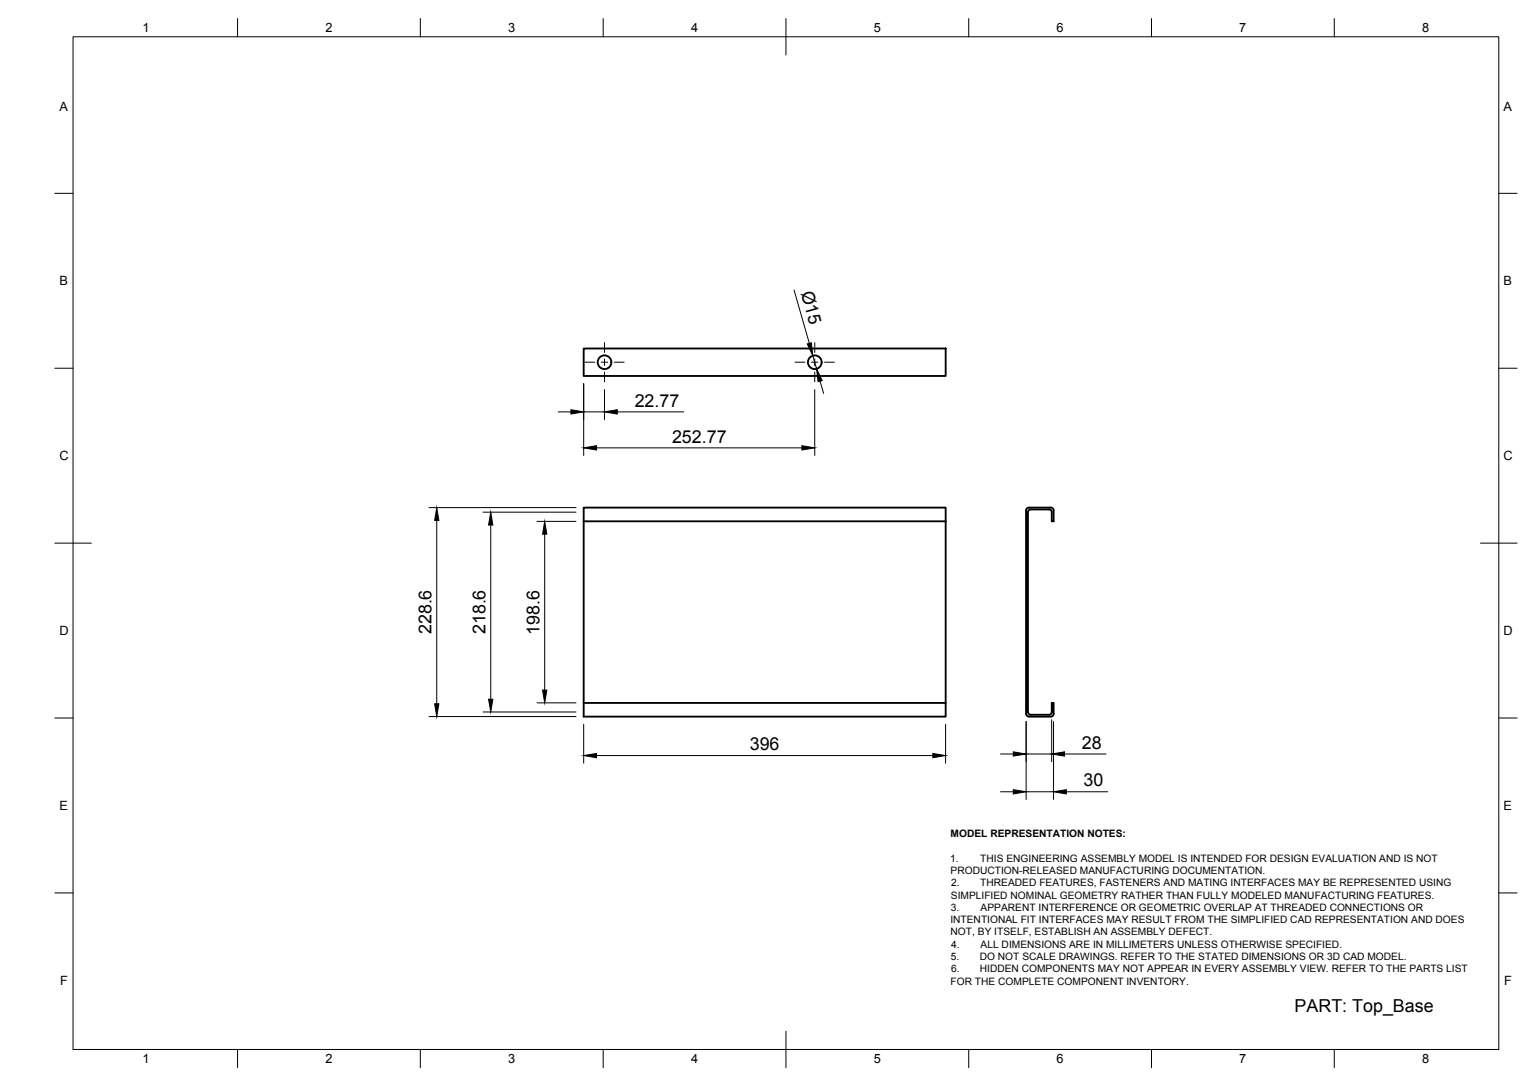
ISO-10303-21;
HEADER;
/* Generated by software containing ST-Developer
 * from STEP Tools, Inc. (www.steptools.com) 
 */

FILE_DESCRIPTION(
/* description */ (''),
/* implementation_level */ '2;1');

FILE_NAME(
/* name */ 'Top_Base.step',
/* time_stamp */ '2026-10-05T15:35:09-07:00',
/* author */ (''),
/* organization */ (''),
/* preprocessor_version */ 'ST-DEVELOPER v20.2',
/* originating_system */ 'Autodesk Translation Framework v15.15.0.0',
/* authorisation */ '');

FILE_SCHEMA (('AUTOMOTIVE_DESIGN { 1 0 10303 214 3 1 1 }'));
ENDSEC;

DATA;
#10=MECHANICAL_DESIGN_GEOMETRIC_PRESENTATION_REPRESENTATION('',(#548),#74523);
#530=SHAPE_REPRESENTATION_RELATIONSHIP('SRR','None',#74563,#539);
#539=ADVANCED_BREP_SHAPE_REPRESENTATION('',(#557),#74519);
#548=STYLED_ITEM('',(#74612),#557);
#557=MANIFOLD_SOLID_BREP('Body1',#4727);
#594=FACE_BOUND('',#944,.T.);
#595=FACE_BOUND('',#945,.T.);
#596=FACE_BOUND('',#949,.T.);
#597=FACE_BOUND('',#950,.T.);
#598=FACE_BOUND('',#958,.T.);
#599=FACE_BOUND('',#959,.T.);
#600=FACE_BOUND('',#965,.T.);
#601=FACE_BOUND('',#966,.T.);
#649=PLANE('',#4999);
#650=PLANE('',#5000);
#651=PLANE('',#5004);
#652=PLANE('',#5011);
#653=PLANE('',#5015);
#654=PLANE('',#5016);
#655=PLANE('',#5021);
#656=PLANE('',#5022);
#657=PLANE('',#5025);
#658=PLANE('',#5028);
#659=PLANE('',#5029);
#660=PLANE('',#5032);
#661=PLANE('',#5035);
#662=PLANE('',#5036);
#759=FACE_OUTER_BOUND('',#936,.T.);
#760=FACE_OUTER_BOUND('',#937,.T.);
#761=FACE_OUTER_BOUND('',#938,.T.);
#762=FACE_OUTER_BOUND('',#939,.T.);
#763=FACE_OUTER_BOUND('',#940,.T.);
#764=FACE_OUTER_BOUND('',#941,.T.);
#765=FACE_OUTER_BOUND('',#942,.T.);
#766=FACE_OUTER_BOUND('',#943,.T.);
#767=FACE_OUTER_BOUND('',#946,.T.);
#768=FACE_OUTER_BOUND('',#947,.T.);
#769=FACE_OUTER_BOUND('',#948,.T.);
#770=FACE_OUTER_BOUND('',#951,.T.);
#771=FACE_OUTER_BOUND('',#952,.T.);
#772=FACE_OUTER_BOUND('',#953,.T.);
#773=FACE_OUTER_BOUND('',#954,.T.);
#774=FACE_OUTER_BOUND('',#955,.T.);
#775=FACE_OUTER_BOUND('',#956,.T.);
#776=FACE_OUTER_BOUND('',#957,.T.);
#777=FACE_OUTER_BOUND('',#960,.T.);
#778=FACE_OUTER_BOUND('',#961,.T.);
#779=FACE_OUTER_BOUND('',#962,.T.);
#780=FACE_OUTER_BOUND('',#963,.T.);
#781=FACE_OUTER_BOUND('',#964,.T.);
#782=FACE_OUTER_BOUND('',#967,.T.);
#783=FACE_OUTER_BOUND('',#968,.T.);
#784=FACE_OUTER_BOUND('',#969,.T.);
#936=EDGE_LOOP('',(#3332,#3333,#3334,#3335));
#937=EDGE_LOOP('',(#3336,#3337,#3338,#3339));
#938=EDGE_LOOP('',(#3340,#3341,#3342,#3343));
#939=EDGE_LOOP('',(#3344,#3345,#3346,#3347));
#940=EDGE_LOOP('',(#3348,#3349,#3350,#3351));
#941=EDGE_LOOP('',(#3352,#3353,#3354,#3355));
#942=EDGE_LOOP('',(#3356,#3357,#3358,#3359));
#943=EDGE_LOOP('',(#3360,#3361,#3362,#3363));
#944=EDGE_LOOP('',(#3364));
#945=EDGE_LOOP('',(#3365));
#946=EDGE_LOOP('',(#3366,#3367,#3368,#3369));
#947=EDGE_LOOP('',(#3370,#3371,#3372,#3373));
#948=EDGE_LOOP('',(#3374,#3375,#3376,#3377));
#949=EDGE_LOOP('',(#3378));
#950=EDGE_LOOP('',(#3379));
#951=EDGE_LOOP('',(#3380,#3381,#3382,#3383));
#952=EDGE_LOOP('',(#3384,#3385,#3386,#3387));
#953=EDGE_LOOP('',(#3388,#3389,#3390,#3391,#3392,#3393,#3394,#3395,#3396,
#3397,#3398,#3399,#3400,#3401,#3402,#3403,#3404,#3405,#3406,#3407));
#954=EDGE_LOOP('',(#3408,#3409,#3410,#3411));
#955=EDGE_LOOP('',(#3412,#3413,#3414,#3415));
#956=EDGE_LOOP('',(#3416,#3417,#3418,#3419));
#957=EDGE_LOOP('',(#3420,#3421,#3422,#3423));
#958=EDGE_LOOP('',(#3424));
#959=EDGE_LOOP('',(#3425));
#960=EDGE_LOOP('',(#3426,#3427,#3428,#3429));
#961=EDGE_LOOP('',(#3430,#3431,#3432,#3433));
#962=EDGE_LOOP('',(#3434,#3435,#3436,#3437));
#963=EDGE_LOOP('',(#3438,#3439,#3440,#3441));
#964=EDGE_LOOP('',(#3442,#3443,#3444,#3445));
#965=EDGE_LOOP('',(#3446));
#966=EDGE_LOOP('',(#3447));
#967=EDGE_LOOP('',(#3448,#3449,#3450,#3451));
#968=EDGE_LOOP('',(#3452,#3453,#3454,#3455));
#969=EDGE_LOOP('',(#3456,#3457,#3458,#3459,#3460,#3461,#3462,#3463,#3464,
#3465,#3466,#3467,#3468,#3469,#3470,#3471,#3472,#3473,#3474,#3475));
#1128=LINE('',#6314,#1325);
#1129=LINE('',#6320,#1326);
#1130=LINE('',#6326,#1327);
#1131=LINE('',#6332,#1328);
#1132=LINE('',#6337,#1329);
#1133=LINE('',#6339,#1330);
#1134=LINE('',#6341,#1331);
#1135=LINE('',#6342,#1332);
#1136=LINE('',#6345,#1333);
#1137=LINE('',#6347,#1334);
#1138=LINE('',#6348,#1335);
#1139=LINE('',#6353,#1336);
#1140=LINE('',#6357,#1337);
#1141=LINE('',#6359,#1338);
#1142=LINE('',#6360,#1339);
#1143=LINE('',#6365,#1340);
#1144=LINE('',#6370,#1341);
#1145=LINE('',#6374,#1342);
#1146=LINE('',#6378,#1343);
#1147=LINE('',#6380,#1344);
#1148=LINE('',#6381,#1345);
#1149=LINE('',#6386,#1346);
#1150=LINE('',#6389,#1347);
#1151=LINE('',#6390,#1348);
#1152=LINE('',#6394,#1349);
#1153=LINE('',#6396,#1350);
#1154=LINE('',#6398,#1351);
#1155=LINE('',#6402,#1352);
#1156=LINE('',#6405,#1353);
#1157=LINE('',#6407,#1354);
#1158=LINE('',#6411,#1355);
#1159=LINE('',#6415,#1356);
#1160=LINE('',#6417,#1357);
#1161=LINE('',#6418,#1358);
#1162=LINE('',#6421,#1359);
#1163=LINE('',#6422,#1360);
#1164=LINE('',#6426,#1361);
#1165=LINE('',#6429,#1362);
#1166=LINE('',#6430,#1363);
#1167=LINE('',#6434,#1364);
#1168=LINE('',#6436,#1365);
#1169=LINE('',#6439,#1366);
#1170=LINE('',#6440,#1367);
#1171=LINE('',#6444,#1368);
#1172=LINE('',#6447,#1369);
#1173=LINE('',#6448,#1370);
#1174=LINE('',#6452,#1371);
#1175=LINE('',#6454,#1372);
#1325=VECTOR('',#5524,7.5);
#1326=VECTOR('',#5531,7.5);
#1327=VECTOR('',#5538,7.5);
#1328=VECTOR('',#5545,7.5);
#1329=VECTOR('',#5550,10.);
#1330=VECTOR('',#5551,10.);
#1331=VECTOR('',#5552,10.);
#1332=VECTOR('',#5553,10.);
#1333=VECTOR('',#5556,10.);
#1334=VECTOR('',#5557,10.);
#1335=VECTOR('',#5558,10.);
#1336=VECTOR('',#5563,10.);
#1337=VECTOR('',#5568,10.);
#1338=VECTOR('',#5569,10.);
#1339=VECTOR('',#5570,10.);
#1340=VECTOR('',#5575,10.);
#1341=VECTOR('',#5580,10.);
#1342=VECTOR('',#5583,10.);
#1343=VECTOR('',#5588,10.);
#1344=VECTOR('',#5589,10.);
#1345=VECTOR('',#5590,10.);
#1346=VECTOR('',#5595,10.);
#1347=VECTOR('',#5600,10.);
#1348=VECTOR('',#5601,10.);
#1349=VECTOR('',#5604,10.);
#1350=VECTOR('',#5605,10.);
#1351=VECTOR('',#5606,10.);
#1352=VECTOR('',#5609,10.);
#1353=VECTOR('',#5612,10.);
#1354=VECTOR('',#5613,10.);
#1355=VECTOR('',#5616,10.);
#1356=VECTOR('',#5621,10.);
#1357=VECTOR('',#5622,10.);
#1358=VECTOR('',#5623,10.);
#1359=VECTOR('',#5626,10.);
#1360=VECTOR('',#5627,10.);
#1361=VECTOR('',#5632,10.);
#1362=VECTOR('',#5635,10.);
#1363=VECTOR('',#5636,10.);
#1364=VECTOR('',#5641,10.);
#1365=VECTOR('',#5644,10.);
#1366=VECTOR('',#5647,10.);
#1367=VECTOR('',#5648,10.);
#1368=VECTOR('',#5653,10.);
#1369=VECTOR('',#5656,10.);
#1370=VECTOR('',#5657,10.);
#1371=VECTOR('',#5662,10.);
#1372=VECTOR('',#5665,10.);
#1484=CIRCLE('',#4988,7.5);
#1485=CIRCLE('',#4989,7.5);
#1486=CIRCLE('',#4991,7.5);
#1487=CIRCLE('',#4992,7.5);
#1488=CIRCLE('',#4994,7.5);
#1489=CIRCLE('',#4995,7.5);
#1490=CIRCLE('',#4997,7.5);
#1491=CIRCLE('',#4998,7.5);
#1492=CIRCLE('',#5002,3.00000000000002);
#1493=CIRCLE('',#5003,3.00000000000002);
#1494=CIRCLE('',#5006,3.00000000000002);
#1495=CIRCLE('',#5007,3.00000000000002);
#1496=CIRCLE('',#5009,3.00000000000002);
#1497=CIRCLE('',#5010,3.00000000000002);
#1498=CIRCLE('',#5013,3.00000000000002);
#1499=CIRCLE('',#5014,3.00000000000002);
#1500=CIRCLE('',#5017,3.00000000000002);
#1501=CIRCLE('',#5018,3.00000000000002);
#1502=CIRCLE('',#5019,3.00000000000002);
#1503=CIRCLE('',#5020,3.00000000000002);
#1504=CIRCLE('',#5024,3.00000000000002);
#1505=CIRCLE('',#5027,3.00000000000002);
#1506=CIRCLE('',#5031,3.00000000000002);
#1507=CIRCLE('',#5034,3.00000000000002);
#1647=VERTEX_POINT('',#6311);
#1648=VERTEX_POINT('',#6313);
#1649=VERTEX_POINT('',#6317);
#1650=VERTEX_POINT('',#6319);
#1651=VERTEX_POINT('',#6323);
#1652=VERTEX_POINT('',#6325);
#1653=VERTEX_POINT('',#6329);
#1654=VERTEX_POINT('',#6331);
#1655=VERTEX_POINT('',#6335);
#1656=VERTEX_POINT('',#6336);
#1657=VERTEX_POINT('',#6338);
#1658=VERTEX_POINT('',#6340);
#1659=VERTEX_POINT('',#6344);
#1660=VERTEX_POINT('',#6346);
#1661=VERTEX_POINT('',#6350);
#1662=VERTEX_POINT('',#6352);
#1663=VERTEX_POINT('',#6356);
#1664=VERTEX_POINT('',#6358);
#1665=VERTEX_POINT('',#6362);
#1666=VERTEX_POINT('',#6364);
#1667=VERTEX_POINT('',#6368);
#1668=VERTEX_POINT('',#6369);
#1669=VERTEX_POINT('',#6371);
#1670=VERTEX_POINT('',#6373);
#1671=VERTEX_POINT('',#6377);
#1672=VERTEX_POINT('',#6379);
#1673=VERTEX_POINT('',#6383);
#1674=VERTEX_POINT('',#6385);
#1675=VERTEX_POINT('',#6392);
#1676=VERTEX_POINT('',#6393);
#1677=VERTEX_POINT('',#6395);
#1678=VERTEX_POINT('',#6397);
#1679=VERTEX_POINT('',#6399);
#1680=VERTEX_POINT('',#6401);
#1681=VERTEX_POINT('',#6403);
#1682=VERTEX_POINT('',#6406);
#1683=VERTEX_POINT('',#6408);
#1684=VERTEX_POINT('',#6410);
#1685=VERTEX_POINT('',#6414);
#1686=VERTEX_POINT('',#6416);
#1687=VERTEX_POINT('',#6420);
#1688=VERTEX_POINT('',#6424);
#1689=VERTEX_POINT('',#6428);
#1690=VERTEX_POINT('',#6432);
#1691=VERTEX_POINT('',#6438);
#1692=VERTEX_POINT('',#6442);
#1693=VERTEX_POINT('',#6446);
#1694=VERTEX_POINT('',#6450);
#2367=EDGE_CURVE('',#1647,#1647,#1484,.T.);
#2368=EDGE_CURVE('',#1647,#1648,#1128,.T.);
#2369=EDGE_CURVE('',#1648,#1648,#1485,.T.);
#2370=EDGE_CURVE('',#1649,#1649,#1486,.T.);
#2371=EDGE_CURVE('',#1649,#1650,#1129,.T.);
#2372=EDGE_CURVE('',#1650,#1650,#1487,.T.);
#2373=EDGE_CURVE('',#1651,#1651,#1488,.T.);
#2374=EDGE_CURVE('',#1651,#1652,#1130,.T.);
#2375=EDGE_CURVE('',#1652,#1652,#1489,.T.);
#2376=EDGE_CURVE('',#1653,#1653,#1490,.T.);
#2377=EDGE_CURVE('',#1653,#1654,#1131,.T.);
#2378=EDGE_CURVE('',#1654,#1654,#1491,.T.);
#2379=EDGE_CURVE('',#1655,#1656,#1132,.T.);
#2380=EDGE_CURVE('',#1656,#1657,#1133,.T.);
#2381=EDGE_CURVE('',#1657,#1658,#1134,.T.);
#2382=EDGE_CURVE('',#1658,#1655,#1135,.T.);
#2383=EDGE_CURVE('',#1657,#1659,#1136,.T.);
#2384=EDGE_CURVE('',#1659,#1660,#1137,.T.);
#2385=EDGE_CURVE('',#1660,#1658,#1138,.T.);
#2386=EDGE_CURVE('',#1659,#1661,#1492,.T.);
#2387=EDGE_CURVE('',#1661,#1662,#1139,.T.);
#2388=EDGE_CURVE('',#1662,#1660,#1493,.T.);
#2389=EDGE_CURVE('',#1661,#1663,#1140,.T.);
#2390=EDGE_CURVE('',#1663,#1664,#1141,.T.);
#2391=EDGE_CURVE('',#1664,#1662,#1142,.T.);
#2392=EDGE_CURVE('',#1663,#1665,#1494,.T.);
#2393=EDGE_CURVE('',#1665,#1666,#1143,.T.);
#2394=EDGE_CURVE('',#1666,#1664,#1495,.T.);
#2395=EDGE_CURVE('',#1667,#1668,#1144,.T.);
#2396=EDGE_CURVE('',#1667,#1669,#1496,.T.);
#2397=EDGE_CURVE('',#1669,#1670,#1145,.T.);
#2398=EDGE_CURVE('',#1670,#1668,#1497,.T.);
#2399=EDGE_CURVE('',#1669,#1671,#1146,.T.);
#2400=EDGE_CURVE('',#1671,#1672,#1147,.T.);
#2401=EDGE_CURVE('',#1672,#1670,#1148,.T.);
#2402=EDGE_CURVE('',#1671,#1673,#1498,.T.);
#2403=EDGE_CURVE('',#1673,#1674,#1149,.T.);
#2404=EDGE_CURVE('',#1674,#1672,#1499,.T.);
#2405=EDGE_CURVE('',#1673,#1656,#1150,.T.);
#2406=EDGE_CURVE('',#1655,#1674,#1151,.T.);
#2407=EDGE_CURVE('',#1675,#1676,#1152,.T.);
#2408=EDGE_CURVE('',#1676,#1677,#1153,.T.);
#2409=EDGE_CURVE('',#1677,#1678,#1154,.T.);
#2410=EDGE_CURVE('',#1678,#1679,#1500,.T.);
#2411=EDGE_CURVE('',#1679,#1680,#1155,.T.);
#2412=EDGE_CURVE('',#1680,#1681,#1501,.T.);
#2413=EDGE_CURVE('',#1681,#1665,#1156,.T.);
#2414=EDGE_CURVE('',#1682,#1667,#1157,.T.);
#2415=EDGE_CURVE('',#1682,#1683,#1502,.T.);
#2416=EDGE_CURVE('',#1683,#1684,#1158,.T.);
#2417=EDGE_CURVE('',#1684,#1675,#1503,.T.);
#2418=EDGE_CURVE('',#1685,#1676,#1159,.T.);
#2419=EDGE_CURVE('',#1686,#1685,#1160,.T.);
#2420=EDGE_CURVE('',#1677,#1686,#1161,.T.);
#2421=EDGE_CURVE('',#1687,#1686,#1162,.T.);
#2422=EDGE_CURVE('',#1678,#1687,#1163,.T.);
#2423=EDGE_CURVE('',#1688,#1687,#1504,.T.);
#2424=EDGE_CURVE('',#1679,#1688,#1164,.T.);
#2425=EDGE_CURVE('',#1689,#1688,#1165,.T.);
#2426=EDGE_CURVE('',#1680,#1689,#1166,.T.);
#2427=EDGE_CURVE('',#1690,#1689,#1505,.T.);
#2428=EDGE_CURVE('',#1681,#1690,#1167,.T.);
#2429=EDGE_CURVE('',#1690,#1666,#1168,.T.);
#2430=EDGE_CURVE('',#1691,#1668,#1169,.T.);
#2431=EDGE_CURVE('',#1682,#1691,#1170,.T.);
#2432=EDGE_CURVE('',#1692,#1691,#1506,.T.);
#2433=EDGE_CURVE('',#1683,#1692,#1171,.T.);
#2434=EDGE_CURVE('',#1693,#1692,#1172,.T.);
#2435=EDGE_CURVE('',#1684,#1693,#1173,.T.);
#2436=EDGE_CURVE('',#1694,#1693,#1507,.T.);
#2437=EDGE_CURVE('',#1675,#1694,#1174,.T.);
#2438=EDGE_CURVE('',#1685,#1694,#1175,.T.);
#3332=ORIENTED_EDGE('',*,*,#2367,.F.);
#3333=ORIENTED_EDGE('',*,*,#2368,.T.);
#3334=ORIENTED_EDGE('',*,*,#2369,.F.);
#3335=ORIENTED_EDGE('',*,*,#2368,.F.);
#3336=ORIENTED_EDGE('',*,*,#2370,.F.);
#3337=ORIENTED_EDGE('',*,*,#2371,.T.);
#3338=ORIENTED_EDGE('',*,*,#2372,.F.);
#3339=ORIENTED_EDGE('',*,*,#2371,.F.);
#3340=ORIENTED_EDGE('',*,*,#2373,.F.);
#3341=ORIENTED_EDGE('',*,*,#2374,.T.);
#3342=ORIENTED_EDGE('',*,*,#2375,.F.);
#3343=ORIENTED_EDGE('',*,*,#2374,.F.);
#3344=ORIENTED_EDGE('',*,*,#2376,.F.);
#3345=ORIENTED_EDGE('',*,*,#2377,.T.);
#3346=ORIENTED_EDGE('',*,*,#2378,.F.);
#3347=ORIENTED_EDGE('',*,*,#2377,.F.);
#3348=ORIENTED_EDGE('',*,*,#2379,.T.);
#3349=ORIENTED_EDGE('',*,*,#2380,.T.);
#3350=ORIENTED_EDGE('',*,*,#2381,.T.);
#3351=ORIENTED_EDGE('',*,*,#2382,.T.);
#3352=ORIENTED_EDGE('',*,*,#2381,.F.);
#3353=ORIENTED_EDGE('',*,*,#2383,.T.);
#3354=ORIENTED_EDGE('',*,*,#2384,.T.);
#3355=ORIENTED_EDGE('',*,*,#2385,.T.);
#3356=ORIENTED_EDGE('',*,*,#2384,.F.);
#3357=ORIENTED_EDGE('',*,*,#2386,.T.);
#3358=ORIENTED_EDGE('',*,*,#2387,.T.);
#3359=ORIENTED_EDGE('',*,*,#2388,.T.);
#3360=ORIENTED_EDGE('',*,*,#2387,.F.);
#3361=ORIENTED_EDGE('',*,*,#2389,.T.);
#3362=ORIENTED_EDGE('',*,*,#2390,.T.);
#3363=ORIENTED_EDGE('',*,*,#2391,.T.);
#3364=ORIENTED_EDGE('',*,*,#2370,.T.);
#3365=ORIENTED_EDGE('',*,*,#2376,.T.);
#3366=ORIENTED_EDGE('',*,*,#2390,.F.);
#3367=ORIENTED_EDGE('',*,*,#2392,.T.);
#3368=ORIENTED_EDGE('',*,*,#2393,.T.);
#3369=ORIENTED_EDGE('',*,*,#2394,.T.);
#3370=ORIENTED_EDGE('',*,*,#2395,.F.);
#3371=ORIENTED_EDGE('',*,*,#2396,.T.);
#3372=ORIENTED_EDGE('',*,*,#2397,.T.);
#3373=ORIENTED_EDGE('',*,*,#2398,.T.);
#3374=ORIENTED_EDGE('',*,*,#2397,.F.);
#3375=ORIENTED_EDGE('',*,*,#2399,.T.);
#3376=ORIENTED_EDGE('',*,*,#2400,.T.);
#3377=ORIENTED_EDGE('',*,*,#2401,.T.);
#3378=ORIENTED_EDGE('',*,*,#2372,.T.);
#3379=ORIENTED_EDGE('',*,*,#2378,.T.);
#3380=ORIENTED_EDGE('',*,*,#2400,.F.);
#3381=ORIENTED_EDGE('',*,*,#2402,.T.);
#3382=ORIENTED_EDGE('',*,*,#2403,.T.);
#3383=ORIENTED_EDGE('',*,*,#2404,.T.);
#3384=ORIENTED_EDGE('',*,*,#2403,.F.);
#3385=ORIENTED_EDGE('',*,*,#2405,.T.);
#3386=ORIENTED_EDGE('',*,*,#2379,.F.);
#3387=ORIENTED_EDGE('',*,*,#2406,.T.);
#3388=ORIENTED_EDGE('',*,*,#2407,.T.);
#3389=ORIENTED_EDGE('',*,*,#2408,.T.);
#3390=ORIENTED_EDGE('',*,*,#2409,.T.);
#3391=ORIENTED_EDGE('',*,*,#2410,.T.);
#3392=ORIENTED_EDGE('',*,*,#2411,.T.);
#3393=ORIENTED_EDGE('',*,*,#2412,.T.);
#3394=ORIENTED_EDGE('',*,*,#2413,.T.);
#3395=ORIENTED_EDGE('',*,*,#2392,.F.);
#3396=ORIENTED_EDGE('',*,*,#2389,.F.);
#3397=ORIENTED_EDGE('',*,*,#2386,.F.);
#3398=ORIENTED_EDGE('',*,*,#2383,.F.);
#3399=ORIENTED_EDGE('',*,*,#2380,.F.);
#3400=ORIENTED_EDGE('',*,*,#2405,.F.);
#3401=ORIENTED_EDGE('',*,*,#2402,.F.);
#3402=ORIENTED_EDGE('',*,*,#2399,.F.);
#3403=ORIENTED_EDGE('',*,*,#2396,.F.);
#3404=ORIENTED_EDGE('',*,*,#2414,.F.);
#3405=ORIENTED_EDGE('',*,*,#2415,.T.);
#3406=ORIENTED_EDGE('',*,*,#2416,.T.);
#3407=ORIENTED_EDGE('',*,*,#2417,.T.);
#3408=ORIENTED_EDGE('',*,*,#2418,.F.);
#3409=ORIENTED_EDGE('',*,*,#2419,.F.);
#3410=ORIENTED_EDGE('',*,*,#2420,.F.);
#3411=ORIENTED_EDGE('',*,*,#2408,.F.);
#3412=ORIENTED_EDGE('',*,*,#2420,.T.);
#3413=ORIENTED_EDGE('',*,*,#2421,.F.);
#3414=ORIENTED_EDGE('',*,*,#2422,.F.);
#3415=ORIENTED_EDGE('',*,*,#2409,.F.);
#3416=ORIENTED_EDGE('',*,*,#2422,.T.);
#3417=ORIENTED_EDGE('',*,*,#2423,.F.);
#3418=ORIENTED_EDGE('',*,*,#2424,.F.);
#3419=ORIENTED_EDGE('',*,*,#2410,.F.);
#3420=ORIENTED_EDGE('',*,*,#2424,.T.);
#3421=ORIENTED_EDGE('',*,*,#2425,.F.);
#3422=ORIENTED_EDGE('',*,*,#2426,.F.);
#3423=ORIENTED_EDGE('',*,*,#2411,.F.);
#3424=ORIENTED_EDGE('',*,*,#2369,.T.);
#3425=ORIENTED_EDGE('',*,*,#2375,.T.);
#3426=ORIENTED_EDGE('',*,*,#2426,.T.);
#3427=ORIENTED_EDGE('',*,*,#2427,.F.);
#3428=ORIENTED_EDGE('',*,*,#2428,.F.);
#3429=ORIENTED_EDGE('',*,*,#2412,.F.);
#3430=ORIENTED_EDGE('',*,*,#2428,.T.);
#3431=ORIENTED_EDGE('',*,*,#2429,.T.);
#3432=ORIENTED_EDGE('',*,*,#2393,.F.);
#3433=ORIENTED_EDGE('',*,*,#2413,.F.);
#3434=ORIENTED_EDGE('',*,*,#2430,.F.);
#3435=ORIENTED_EDGE('',*,*,#2431,.F.);
#3436=ORIENTED_EDGE('',*,*,#2414,.T.);
#3437=ORIENTED_EDGE('',*,*,#2395,.T.);
#3438=ORIENTED_EDGE('',*,*,#2431,.T.);
#3439=ORIENTED_EDGE('',*,*,#2432,.F.);
#3440=ORIENTED_EDGE('',*,*,#2433,.F.);
#3441=ORIENTED_EDGE('',*,*,#2415,.F.);
#3442=ORIENTED_EDGE('',*,*,#2433,.T.);
#3443=ORIENTED_EDGE('',*,*,#2434,.F.);
#3444=ORIENTED_EDGE('',*,*,#2435,.F.);
#3445=ORIENTED_EDGE('',*,*,#2416,.F.);
#3446=ORIENTED_EDGE('',*,*,#2367,.T.);
#3447=ORIENTED_EDGE('',*,*,#2373,.T.);
#3448=ORIENTED_EDGE('',*,*,#2435,.T.);
#3449=ORIENTED_EDGE('',*,*,#2436,.F.);
#3450=ORIENTED_EDGE('',*,*,#2437,.F.);
#3451=ORIENTED_EDGE('',*,*,#2417,.F.);
#3452=ORIENTED_EDGE('',*,*,#2437,.T.);
#3453=ORIENTED_EDGE('',*,*,#2438,.F.);
#3454=ORIENTED_EDGE('',*,*,#2418,.T.);
#3455=ORIENTED_EDGE('',*,*,#2407,.F.);
#3456=ORIENTED_EDGE('',*,*,#2438,.T.);
#3457=ORIENTED_EDGE('',*,*,#2436,.T.);
#3458=ORIENTED_EDGE('',*,*,#2434,.T.);
#3459=ORIENTED_EDGE('',*,*,#2432,.T.);
#3460=ORIENTED_EDGE('',*,*,#2430,.T.);
#3461=ORIENTED_EDGE('',*,*,#2398,.F.);
#3462=ORIENTED_EDGE('',*,*,#2401,.F.);
#3463=ORIENTED_EDGE('',*,*,#2404,.F.);
#3464=ORIENTED_EDGE('',*,*,#2406,.F.);
#3465=ORIENTED_EDGE('',*,*,#2382,.F.);
#3466=ORIENTED_EDGE('',*,*,#2385,.F.);
#3467=ORIENTED_EDGE('',*,*,#2388,.F.);
#3468=ORIENTED_EDGE('',*,*,#2391,.F.);
#3469=ORIENTED_EDGE('',*,*,#2394,.F.);
#3470=ORIENTED_EDGE('',*,*,#2429,.F.);
#3471=ORIENTED_EDGE('',*,*,#2427,.T.);
#3472=ORIENTED_EDGE('',*,*,#2425,.T.);
#3473=ORIENTED_EDGE('',*,*,#2423,.T.);
#3474=ORIENTED_EDGE('',*,*,#2421,.T.);
#3475=ORIENTED_EDGE('',*,*,#2419,.T.);
#4551=CYLINDRICAL_SURFACE('',#4987,7.5);
#4552=CYLINDRICAL_SURFACE('',#4990,7.5);
#4553=CYLINDRICAL_SURFACE('',#4993,7.5);
#4554=CYLINDRICAL_SURFACE('',#4996,7.5);
#4555=CYLINDRICAL_SURFACE('',#5001,3.00000000000002);
#4556=CYLINDRICAL_SURFACE('',#5005,3.00000000000002);
#4557=CYLINDRICAL_SURFACE('',#5008,3.00000000000002);
#4558=CYLINDRICAL_SURFACE('',#5012,3.00000000000002);
#4559=CYLINDRICAL_SURFACE('',#5023,3.00000000000002);
#4560=CYLINDRICAL_SURFACE('',#5026,3.00000000000002);
#4561=CYLINDRICAL_SURFACE('',#5030,3.00000000000002);
#4562=CYLINDRICAL_SURFACE('',#5033,3.00000000000002);
#4655=ADVANCED_FACE('',(#759),#4551,.F.);
#4656=ADVANCED_FACE('',(#760),#4552,.F.);
#4657=ADVANCED_FACE('',(#761),#4553,.F.);
#4658=ADVANCED_FACE('',(#762),#4554,.F.);
#4659=ADVANCED_FACE('',(#763),#649,.F.);
#4660=ADVANCED_FACE('',(#764),#650,.F.);
#4661=ADVANCED_FACE('',(#765),#4555,.F.);
#4662=ADVANCED_FACE('',(#766,#594,#595),#651,.F.);
#4663=ADVANCED_FACE('',(#767),#4556,.F.);
#4664=ADVANCED_FACE('',(#768),#4557,.T.);
#4665=ADVANCED_FACE('',(#769,#596,#597),#652,.F.);
#4666=ADVANCED_FACE('',(#770),#4558,.T.);
#4667=ADVANCED_FACE('',(#771),#653,.F.);
#4668=ADVANCED_FACE('',(#772),#654,.F.);
#4669=ADVANCED_FACE('',(#773),#655,.T.);
#4670=ADVANCED_FACE('',(#774),#656,.T.);
#4671=ADVANCED_FACE('',(#775),#4559,.F.);
#4672=ADVANCED_FACE('',(#776,#598,#599),#657,.T.);
#4673=ADVANCED_FACE('',(#777),#4560,.F.);
#4674=ADVANCED_FACE('',(#778),#658,.T.);
#4675=ADVANCED_FACE('',(#779),#659,.T.);
#4676=ADVANCED_FACE('',(#780),#4561,.T.);
#4677=ADVANCED_FACE('',(#781,#600,#601),#660,.T.);
#4678=ADVANCED_FACE('',(#782),#4562,.T.);
#4679=ADVANCED_FACE('',(#783),#661,.T.);
#4680=ADVANCED_FACE('',(#784),#662,.T.);
#4727=CLOSED_SHELL('',(#4655,#4656,#4657,#4658,#4659,#4660,#4661,#4662,
#4663,#4664,#4665,#4666,#4667,#4668,#4669,#4670,#4671,#4672,#4673,#4674,
#4675,#4676,#4677,#4678,#4679,#4680));
#4986=AXIS2_PLACEMENT_3D('',#6309,#5518,#5519);
#4987=AXIS2_PLACEMENT_3D('',#6310,#5520,#5521);
#4988=AXIS2_PLACEMENT_3D('',#6312,#5522,#5523);
#4989=AXIS2_PLACEMENT_3D('',#6315,#5525,#5526);
#4990=AXIS2_PLACEMENT_3D('',#6316,#5527,#5528);
#4991=AXIS2_PLACEMENT_3D('',#6318,#5529,#5530);
#4992=AXIS2_PLACEMENT_3D('',#6321,#5532,#5533);
#4993=AXIS2_PLACEMENT_3D('',#6322,#5534,#5535);
#4994=AXIS2_PLACEMENT_3D('',#6324,#5536,#5537);
#4995=AXIS2_PLACEMENT_3D('',#6327,#5539,#5540);
#4996=AXIS2_PLACEMENT_3D('',#6328,#5541,#5542);
#4997=AXIS2_PLACEMENT_3D('',#6330,#5543,#5544);
#4998=AXIS2_PLACEMENT_3D('',#6333,#5546,#5547);
#4999=AXIS2_PLACEMENT_3D('',#6334,#5548,#5549);
#5000=AXIS2_PLACEMENT_3D('',#6343,#5554,#5555);
#5001=AXIS2_PLACEMENT_3D('',#6349,#5559,#5560);
#5002=AXIS2_PLACEMENT_3D('',#6351,#5561,#5562);
#5003=AXIS2_PLACEMENT_3D('',#6354,#5564,#5565);
#5004=AXIS2_PLACEMENT_3D('',#6355,#5566,#5567);
#5005=AXIS2_PLACEMENT_3D('',#6361,#5571,#5572);
#5006=AXIS2_PLACEMENT_3D('',#6363,#5573,#5574);
#5007=AXIS2_PLACEMENT_3D('',#6366,#5576,#5577);
#5008=AXIS2_PLACEMENT_3D('',#6367,#5578,#5579);
#5009=AXIS2_PLACEMENT_3D('',#6372,#5581,#5582);
#5010=AXIS2_PLACEMENT_3D('',#6375,#5584,#5585);
#5011=AXIS2_PLACEMENT_3D('',#6376,#5586,#5587);
#5012=AXIS2_PLACEMENT_3D('',#6382,#5591,#5592);
#5013=AXIS2_PLACEMENT_3D('',#6384,#5593,#5594);
#5014=AXIS2_PLACEMENT_3D('',#6387,#5596,#5597);
#5015=AXIS2_PLACEMENT_3D('',#6388,#5598,#5599);
#5016=AXIS2_PLACEMENT_3D('',#6391,#5602,#5603);
#5017=AXIS2_PLACEMENT_3D('',#6400,#5607,#5608);
#5018=AXIS2_PLACEMENT_3D('',#6404,#5610,#5611);
#5019=AXIS2_PLACEMENT_3D('',#6409,#5614,#5615);
#5020=AXIS2_PLACEMENT_3D('',#6412,#5617,#5618);
#5021=AXIS2_PLACEMENT_3D('',#6413,#5619,#5620);
#5022=AXIS2_PLACEMENT_3D('',#6419,#5624,#5625);
#5023=AXIS2_PLACEMENT_3D('',#6423,#5628,#5629);
#5024=AXIS2_PLACEMENT_3D('',#6425,#5630,#5631);
#5025=AXIS2_PLACEMENT_3D('',#6427,#5633,#5634);
#5026=AXIS2_PLACEMENT_3D('',#6431,#5637,#5638);
#5027=AXIS2_PLACEMENT_3D('',#6433,#5639,#5640);
#5028=AXIS2_PLACEMENT_3D('',#6435,#5642,#5643);
#5029=AXIS2_PLACEMENT_3D('',#6437,#5645,#5646);
#5030=AXIS2_PLACEMENT_3D('',#6441,#5649,#5650);
#5031=AXIS2_PLACEMENT_3D('',#6443,#5651,#5652);
#5032=AXIS2_PLACEMENT_3D('',#6445,#5654,#5655);
#5033=AXIS2_PLACEMENT_3D('',#6449,#5658,#5659);
#5034=AXIS2_PLACEMENT_3D('',#6451,#5660,#5661);
#5035=AXIS2_PLACEMENT_3D('',#6453,#5663,#5664);
#5036=AXIS2_PLACEMENT_3D('',#6455,#5666,#5667);
#5518=DIRECTION('axis',(0.,0.,1.));
#5519=DIRECTION('refdir',(1.,0.,0.));
#5520=DIRECTION('center_axis',(0.,1.,0.));
#5521=DIRECTION('ref_axis',(1.,0.,0.));
#5522=DIRECTION('center_axis',(0.,1.,0.));
#5523=DIRECTION('ref_axis',(1.,0.,0.));
#5524=DIRECTION('',(0.,1.,0.));
#5525=DIRECTION('center_axis',(-1.08770485875751E-31,-1.,8.88178419700126E-16));
#5526=DIRECTION('ref_axis',(1.,-1.08770485875751E-31,9.66075982551394E-47));
#5527=DIRECTION('center_axis',(0.,1.,0.));
#5528=DIRECTION('ref_axis',(1.,0.,0.));
#5529=DIRECTION('center_axis',(-1.08770485875751E-31,1.,8.88178419700126E-16));
#5530=DIRECTION('ref_axis',(1.,1.08770485875751E-31,9.66075982551394E-47));
#5531=DIRECTION('',(0.,1.,0.));
#5532=DIRECTION('center_axis',(0.,-1.,0.));
#5533=DIRECTION('ref_axis',(1.,0.,0.));
#5534=DIRECTION('center_axis',(0.,1.,0.));
#5535=DIRECTION('ref_axis',(1.,0.,0.));
#5536=DIRECTION('center_axis',(0.,1.,0.));
#5537=DIRECTION('ref_axis',(1.,0.,0.));
#5538=DIRECTION('',(0.,1.,0.));
#5539=DIRECTION('center_axis',(-1.08770485875751E-31,-1.,8.88178419700126E-16));
#5540=DIRECTION('ref_axis',(1.,-1.08770485875751E-31,9.66075982551394E-47));
#5541=DIRECTION('center_axis',(0.,1.,0.));
#5542=DIRECTION('ref_axis',(1.,0.,0.));
#5543=DIRECTION('center_axis',(-1.08770485875751E-31,1.,8.88178419700126E-16));
#5544=DIRECTION('ref_axis',(1.,1.08770485875751E-31,9.66075982551394E-47));
#5545=DIRECTION('',(0.,1.,0.));
#5546=DIRECTION('center_axis',(0.,-1.,0.));
#5547=DIRECTION('ref_axis',(1.,0.,0.));
#5548=DIRECTION('center_axis',(0.,1.,0.));
#5549=DIRECTION('ref_axis',(1.22464679914735E-16,0.,-1.));
#5550=DIRECTION('',(1.,0.,1.22464679914735E-16));
#5551=DIRECTION('',(-1.22464679914735E-16,0.,1.));
#5552=DIRECTION('',(-1.,0.,-1.22464679914735E-16));
#5553=DIRECTION('',(1.22464679914735E-16,0.,-1.));
#5554=DIRECTION('center_axis',(1.22464679914735E-16,0.,-1.));
#5555=DIRECTION('ref_axis',(0.,-1.,0.));
#5556=DIRECTION('',(0.,1.,0.));
#5557=DIRECTION('',(-1.,0.,-1.22464679914735E-16));
#5558=DIRECTION('',(0.,-1.,0.));
#5559=DIRECTION('center_axis',(1.,0.,1.22464679914735E-16));
#5560=DIRECTION('ref_axis',(1.22464679914735E-16,5.92118946466746E-15,-1.));
#5561=DIRECTION('center_axis',(1.,0.,1.22464679914735E-16));
#5562=DIRECTION('ref_axis',(1.22464679914735E-16,5.92118946466746E-15,-1.));
#5563=DIRECTION('',(-1.,0.,-1.22464679914735E-16));
#5564=DIRECTION('center_axis',(-1.,0.,-1.22464679914735E-16));
#5565=DIRECTION('ref_axis',(1.22464679914735E-16,5.92118946466746E-15,-1.));
#5566=DIRECTION('center_axis',(-1.08770485875751E-31,1.,8.88178419700126E-16));
#5567=DIRECTION('ref_axis',(1.22464679914735E-16,8.88178419700126E-16,-1.));
#5568=DIRECTION('',(-1.22464679914735E-16,-8.88178419700126E-16,1.));
#5569=DIRECTION('',(-1.,0.,-1.22464679914735E-16));
#5570=DIRECTION('',(1.22464679914735E-16,8.88178419700126E-16,-1.));
#5571=DIRECTION('center_axis',(1.,0.,1.22464679914735E-16));
#5572=DIRECTION('ref_axis',(-1.0877048587575E-30,1.,8.88178419700118E-15));
#5573=DIRECTION('center_axis',(1.,0.,1.22464679914735E-16));
#5574=DIRECTION('ref_axis',(-1.0877048587575E-30,1.,8.88178419700118E-15));
#5575=DIRECTION('',(-1.,0.,-1.22464679914735E-16));
#5576=DIRECTION('center_axis',(-1.,0.,-1.22464679914735E-16));
#5577=DIRECTION('ref_axis',(-1.0877048587575E-30,1.,8.88178419700118E-15));
#5578=DIRECTION('center_axis',(1.,0.,1.22464679914735E-16));
#5579=DIRECTION('ref_axis',(-9.29081233522032E-31,1.,7.58652400160517E-15));
#5580=DIRECTION('',(-1.,0.,-1.22464679914735E-16));
#5581=DIRECTION('center_axis',(-1.,0.,-1.22464679914735E-16));
#5582=DIRECTION('ref_axis',(-9.29081233522032E-31,1.,7.58652400160517E-15));
#5583=DIRECTION('',(-1.,0.,-1.22464679914735E-16));
#5584=DIRECTION('center_axis',(1.,0.,1.22464679914735E-16));
#5585=DIRECTION('ref_axis',(-9.29081233522032E-31,1.,7.58652400160517E-15));
#5586=DIRECTION('center_axis',(0.,-1.,0.));
#5587=DIRECTION('ref_axis',(-1.22464679914735E-16,0.,1.));
#5588=DIRECTION('',(1.22464679914735E-16,0.,-1.));
#5589=DIRECTION('',(-1.,0.,-1.22464679914735E-16));
#5590=DIRECTION('',(-1.22464679914735E-16,0.,1.));
#5591=DIRECTION('center_axis',(1.,0.,1.22464679914735E-16));
#5592=DIRECTION('ref_axis',(1.22464679914735E-16,5.92118946466745E-15,-1.));
#5593=DIRECTION('center_axis',(-1.,0.,-1.22464679914735E-16));
#5594=DIRECTION('ref_axis',(1.22464679914735E-16,5.92118946466745E-15,-1.));
#5595=DIRECTION('',(-1.,0.,-1.22464679914735E-16));
#5596=DIRECTION('center_axis',(1.,0.,1.22464679914735E-16));
#5597=DIRECTION('ref_axis',(1.22464679914735E-16,5.92118946466745E-15,-1.));
#5598=DIRECTION('center_axis',(-1.22464679914735E-16,0.,1.));
#5599=DIRECTION('ref_axis',(0.,1.,0.));
#5600=DIRECTION('',(0.,-1.,0.));
#5601=DIRECTION('',(0.,1.,0.));
#5602=DIRECTION('center_axis',(-1.,0.,-1.22464679914735E-16));
#5603=DIRECTION('ref_axis',(0.,1.,0.));
#5604=DIRECTION('',(0.,1.,0.));
#5605=DIRECTION('',(-1.22464679914735E-16,0.,1.));
#5606=DIRECTION('',(0.,-1.,0.));
#5607=DIRECTION('center_axis',(-1.,0.,-1.22464679914735E-16));
#5608=DIRECTION('ref_axis',(1.22464679914735E-16,-5.92118946466746E-15,
-1.));
#5609=DIRECTION('',(-1.22464679914735E-16,8.88178419700126E-16,1.));
#5610=DIRECTION('center_axis',(-1.,0.,-1.22464679914735E-16));
#5611=DIRECTION('ref_axis',(-1.0877048587575E-30,-1.,8.88178419700118E-15));
#5612=DIRECTION('',(-9.32958193124582E-34,1.,7.61818177922111E-18));
#5613=DIRECTION('',(-1.83238689143786E-33,1.,1.49625744558646E-17));
#5614=DIRECTION('center_axis',(1.,0.,1.22464679914735E-16));
#5615=DIRECTION('ref_axis',(-9.29081233522032E-31,-1.,7.58652400160517E-15));
#5616=DIRECTION('',(1.22464679914735E-16,0.,-1.));
#5617=DIRECTION('center_axis',(1.,0.,1.22464679914735E-16));
#5618=DIRECTION('ref_axis',(1.22464679914735E-16,-5.92118946466745E-15,
-1.));
#5619=DIRECTION('center_axis',(0.,1.,0.));
#5620=DIRECTION('ref_axis',(1.22464679914735E-16,0.,-1.));
#5621=DIRECTION('',(1.,0.,1.22464679914735E-16));
#5622=DIRECTION('',(1.22464679914735E-16,0.,-1.));
#5623=DIRECTION('',(-1.,0.,-1.22464679914735E-16));
#5624=DIRECTION('center_axis',(-1.22464679914735E-16,0.,1.));
#5625=DIRECTION('ref_axis',(0.,1.,0.));
#5626=DIRECTION('',(0.,1.,0.));
#5627=DIRECTION('',(-1.,0.,-1.22464679914735E-16));
#5628=DIRECTION('center_axis',(-1.,0.,-1.22464679914735E-16));
#5629=DIRECTION('ref_axis',(1.22464679914735E-16,-5.92118946466746E-15,
-1.));
#5630=DIRECTION('center_axis',(1.,0.,1.22464679914735E-16));
#5631=DIRECTION('ref_axis',(1.22464679914735E-16,-5.92118946466746E-15,
-1.));
#5632=DIRECTION('',(-1.,0.,-1.22464679914735E-16));
#5633=DIRECTION('center_axis',(1.08770485875751E-31,1.,-8.88178419700126E-16));
#5634=DIRECTION('ref_axis',(1.22464679914735E-16,-8.88178419700126E-16,
-1.));
#5635=DIRECTION('',(1.22464679914735E-16,-8.88178419700126E-16,-1.));
#5636=DIRECTION('',(-1.,0.,-1.22464679914735E-16));
#5637=DIRECTION('center_axis',(-1.,0.,-1.22464679914735E-16));
#5638=DIRECTION('ref_axis',(-1.0877048587575E-30,-1.,8.88178419700118E-15));
#5639=DIRECTION('center_axis',(1.,0.,1.22464679914735E-16));
#5640=DIRECTION('ref_axis',(-1.0877048587575E-30,-1.,8.88178419700118E-15));
#5641=DIRECTION('',(-1.,0.,-1.22464679914735E-16));
#5642=DIRECTION('center_axis',(1.22464679914735E-16,7.61818177922111E-18,
-1.));
#5643=DIRECTION('ref_axis',(9.32958193124582E-34,-1.,-7.61818177922111E-18));
#5644=DIRECTION('',(9.32958193124582E-34,1.,-7.61818177922111E-18));
#5645=DIRECTION('center_axis',(-1.22464679914735E-16,1.49625744558646E-17,
1.));
#5646=DIRECTION('ref_axis',(1.83238689143786E-33,1.,-1.49625744558646E-17));
#5647=DIRECTION('',(1.83238689143786E-33,1.,-1.49625744558646E-17));
#5648=DIRECTION('',(-1.,0.,-1.22464679914735E-16));
#5649=DIRECTION('center_axis',(-1.,0.,-1.22464679914735E-16));
#5650=DIRECTION('ref_axis',(-9.29081233522032E-31,-1.,7.58652400160517E-15));
#5651=DIRECTION('center_axis',(-1.,0.,-1.22464679914735E-16));
#5652=DIRECTION('ref_axis',(-9.29081233522032E-31,-1.,7.58652400160517E-15));
#5653=DIRECTION('',(-1.,0.,-1.22464679914735E-16));
#5654=DIRECTION('center_axis',(0.,-1.,0.));
#5655=DIRECTION('ref_axis',(-1.22464679914735E-16,0.,1.));
#5656=DIRECTION('',(-1.22464679914735E-16,0.,1.));
#5657=DIRECTION('',(-1.,0.,-1.22464679914735E-16));
#5658=DIRECTION('center_axis',(-1.,0.,-1.22464679914735E-16));
#5659=DIRECTION('ref_axis',(1.22464679914735E-16,-5.92118946466745E-15,
-1.));
#5660=DIRECTION('center_axis',(-1.,0.,-1.22464679914735E-16));
#5661=DIRECTION('ref_axis',(1.22464679914735E-16,-5.92118946466745E-15,
-1.));
#5662=DIRECTION('',(-1.,0.,-1.22464679914735E-16));
#5663=DIRECTION('center_axis',(1.22464679914735E-16,0.,-1.));
#5664=DIRECTION('ref_axis',(0.,-1.,0.));
#5665=DIRECTION('',(0.,-1.,0.));
#5666=DIRECTION('center_axis',(-1.,0.,-1.22464679914735E-16));
#5667=DIRECTION('ref_axis',(0.,1.,0.));
#6309=CARTESIAN_POINT('',(0.,0.,0.));
#6310=CARTESIAN_POINT('Origin',(-54.768323187501,-118.,335.));
#6311=CARTESIAN_POINT('',(-62.268323187501,-114.3,335.));
#6312=CARTESIAN_POINT('Origin',(-54.768323187501,-114.3,335.));
#6313=CARTESIAN_POINT('',(-62.268323187501,-112.3,335.));
#6314=CARTESIAN_POINT('',(-62.268323187501,-118.,335.));
#6315=CARTESIAN_POINT('Origin',(-54.768323187501,-112.3,335.));
#6316=CARTESIAN_POINT('Origin',(-54.768323187501,-118.,335.));
#6317=CARTESIAN_POINT('',(-62.268323187501,112.3,335.));
#6318=CARTESIAN_POINT('Origin',(-54.768323187501,112.3,335.));
#6319=CARTESIAN_POINT('',(-62.268323187501,114.3,335.));
#6320=CARTESIAN_POINT('',(-62.268323187501,-118.,335.));
#6321=CARTESIAN_POINT('Origin',(-54.768323187501,114.3,335.));
#6322=CARTESIAN_POINT('Origin',(175.231676812499,-118.,335.));
#6323=CARTESIAN_POINT('',(167.731676812499,-114.3,335.));
#6324=CARTESIAN_POINT('Origin',(175.231676812499,-114.3,335.));
#6325=CARTESIAN_POINT('',(167.731676812499,-112.3,335.));
#6326=CARTESIAN_POINT('',(167.731676812499,-118.,335.));
#6327=CARTESIAN_POINT('Origin',(175.231676812499,-112.3,335.));
#6328=CARTESIAN_POINT('Origin',(175.231676812499,-118.,335.));
#6329=CARTESIAN_POINT('',(167.731676812499,112.3,335.));
#6330=CARTESIAN_POINT('Origin',(175.231676812499,112.3,335.));
#6331=CARTESIAN_POINT('',(167.731676812499,114.3,335.));
#6332=CARTESIAN_POINT('',(167.731676812499,-118.,335.));
#6333=CARTESIAN_POINT('Origin',(175.231676812499,114.3,335.));
#6334=CARTESIAN_POINT('Origin',(-3.94336269325448E-14,99.3,322.));
#6335=CARTESIAN_POINT('',(-198.,99.3,320.));
#6336=CARTESIAN_POINT('',(198.,99.3,320.));
#6337=CARTESIAN_POINT('',(-3.91886975727153E-14,99.3,320.));
#6338=CARTESIAN_POINT('',(198.,99.3,322.));
#6339=CARTESIAN_POINT('',(198.,99.3,320.));
#6340=CARTESIAN_POINT('',(-198.,99.3,322.));
#6341=CARTESIAN_POINT('',(-3.94336269325448E-14,99.3,322.));
#6342=CARTESIAN_POINT('',(-198.,99.3,320.));
#6343=CARTESIAN_POINT('Origin',(-3.94336269325448E-14,109.3,322.));
#6344=CARTESIAN_POINT('',(198.,109.3,322.));
#6345=CARTESIAN_POINT('',(198.,112.3,322.));
#6346=CARTESIAN_POINT('',(-198.,109.3,322.));
#6347=CARTESIAN_POINT('',(-3.94336269325448E-14,109.3,322.));
#6348=CARTESIAN_POINT('',(-198.,112.3,322.));
#6349=CARTESIAN_POINT('Origin',(-3.9801020972289E-14,109.3,325.));
#6350=CARTESIAN_POINT('',(198.,112.3,325.));
#6351=CARTESIAN_POINT('Origin',(198.,109.3,325.));
#6352=CARTESIAN_POINT('',(-198.,112.3,325.));
#6353=CARTESIAN_POINT('',(-3.9801020972289E-14,112.3,325.));
#6354=CARTESIAN_POINT('Origin',(-198.,109.3,325.));
#6355=CARTESIAN_POINT('Origin',(-4.22503145705837E-14,112.3,345.));
#6356=CARTESIAN_POINT('',(198.,112.3,345.));
#6357=CARTESIAN_POINT('',(198.,112.3,345.));
#6358=CARTESIAN_POINT('',(-198.,112.3,345.));
#6359=CARTESIAN_POINT('',(-4.22503145705837E-14,112.3,345.));
#6360=CARTESIAN_POINT('',(-198.,112.3,345.));
#6361=CARTESIAN_POINT('Origin',(-4.22503145705837E-14,109.3,345.));
#6362=CARTESIAN_POINT('',(198.,109.3,348.));
#6363=CARTESIAN_POINT('Origin',(198.,109.3,345.));
#6364=CARTESIAN_POINT('',(-198.,109.3,348.));
#6365=CARTESIAN_POINT('',(-4.26177086103279E-14,109.3,348.));
#6366=CARTESIAN_POINT('Origin',(-198.,109.3,345.));
#6367=CARTESIAN_POINT('Origin',(-4.24952439304132E-14,111.3,347.));
#6368=CARTESIAN_POINT('',(198.,111.3,350.));
#6369=CARTESIAN_POINT('',(-198.,111.3,350.));
#6370=CARTESIAN_POINT('',(-4.28626379701574E-14,111.3,350.));
#6371=CARTESIAN_POINT('',(198.,114.3,347.));
#6372=CARTESIAN_POINT('Origin',(198.,111.3,347.));
#6373=CARTESIAN_POINT('',(-198.,114.3,347.));
#6374=CARTESIAN_POINT('',(-4.24952439304132E-14,114.3,347.));
#6375=CARTESIAN_POINT('Origin',(-198.,111.3,347.));
#6376=CARTESIAN_POINT('Origin',(-3.95560916124595E-14,114.3,323.));
#6377=CARTESIAN_POINT('',(198.,114.3,323.));
#6378=CARTESIAN_POINT('',(198.,114.3,347.));
#6379=CARTESIAN_POINT('',(-198.,114.3,323.));
#6380=CARTESIAN_POINT('',(-3.95560916124595E-14,114.3,323.));
#6381=CARTESIAN_POINT('',(-198.,114.3,347.));
#6382=CARTESIAN_POINT('Origin',(-3.95560916124595E-14,111.3,323.));
#6383=CARTESIAN_POINT('',(198.,111.3,320.));
#6384=CARTESIAN_POINT('Origin',(198.,111.3,323.));
#6385=CARTESIAN_POINT('',(-198.,111.3,320.));
#6386=CARTESIAN_POINT('',(-3.91886975727153E-14,111.3,320.));
#6387=CARTESIAN_POINT('Origin',(-198.,111.3,323.));
#6388=CARTESIAN_POINT('Origin',(-3.91886975727153E-14,99.3,320.));
#6389=CARTESIAN_POINT('',(198.,111.3,320.));
#6390=CARTESIAN_POINT('',(-198.,111.3,320.));
#6391=CARTESIAN_POINT('Origin',(198.,-57.15,335.));
#6392=CARTESIAN_POINT('',(198.,-111.3,320.));
#6393=CARTESIAN_POINT('',(198.,-99.3,320.));
#6394=CARTESIAN_POINT('',(198.,-111.3,320.));
#6395=CARTESIAN_POINT('',(198.,-99.3,322.));
#6396=CARTESIAN_POINT('',(198.,-99.3,320.));
#6397=CARTESIAN_POINT('',(198.,-109.3,322.));
#6398=CARTESIAN_POINT('',(198.,-112.3,322.));
#6399=CARTESIAN_POINT('',(198.,-112.3,325.));
#6400=CARTESIAN_POINT('Origin',(198.,-109.3,325.));
#6401=CARTESIAN_POINT('',(198.,-112.3,345.));
#6402=CARTESIAN_POINT('',(198.,-112.3,345.));
#6403=CARTESIAN_POINT('',(198.,-109.3,348.));
#6404=CARTESIAN_POINT('Origin',(198.,-109.3,345.));
#6405=CARTESIAN_POINT('',(198.,0.,348.));
#6406=CARTESIAN_POINT('',(198.,-111.3,350.));
#6407=CARTESIAN_POINT('',(198.,0.,350.));
#6408=CARTESIAN_POINT('',(198.,-114.3,347.));
#6409=CARTESIAN_POINT('Origin',(198.,-111.3,347.));
#6410=CARTESIAN_POINT('',(198.,-114.3,323.));
#6411=CARTESIAN_POINT('',(198.,-114.3,347.));
#6412=CARTESIAN_POINT('Origin',(198.,-111.3,323.));
#6413=CARTESIAN_POINT('Origin',(-3.94336269325448E-14,-99.3,322.));
#6414=CARTESIAN_POINT('',(-198.,-99.3,320.));
#6415=CARTESIAN_POINT('',(-3.91886975727153E-14,-99.3,320.));
#6416=CARTESIAN_POINT('',(-198.,-99.3,322.));
#6417=CARTESIAN_POINT('',(-198.,-99.3,320.));
#6418=CARTESIAN_POINT('',(-3.94336269325448E-14,-99.3,322.));
#6419=CARTESIAN_POINT('Origin',(-3.94336269325448E-14,-109.3,322.));
#6420=CARTESIAN_POINT('',(-198.,-109.3,322.));
#6421=CARTESIAN_POINT('',(-198.,-112.3,322.));
#6422=CARTESIAN_POINT('',(-3.94336269325448E-14,-109.3,322.));
#6423=CARTESIAN_POINT('Origin',(-3.9801020972289E-14,-109.3,325.));
#6424=CARTESIAN_POINT('',(-198.,-112.3,325.));
#6425=CARTESIAN_POINT('Origin',(-198.,-109.3,325.));
#6426=CARTESIAN_POINT('',(-3.9801020972289E-14,-112.3,325.));
#6427=CARTESIAN_POINT('Origin',(-4.22503145705837E-14,-112.3,345.));
#6428=CARTESIAN_POINT('',(-198.,-112.3,345.));
#6429=CARTESIAN_POINT('',(-198.,-112.3,345.));
#6430=CARTESIAN_POINT('',(-4.22503145705837E-14,-112.3,345.));
#6431=CARTESIAN_POINT('Origin',(-4.22503145705837E-14,-109.3,345.));
#6432=CARTESIAN_POINT('',(-198.,-109.3,348.));
#6433=CARTESIAN_POINT('Origin',(-198.,-109.3,345.));
#6434=CARTESIAN_POINT('',(-4.26177086103279E-14,-109.3,348.));
#6435=CARTESIAN_POINT('Origin',(-4.26177086103279E-14,0.,348.));
#6436=CARTESIAN_POINT('',(-198.,0.,348.));
#6437=CARTESIAN_POINT('Origin',(-4.28626379701574E-14,-111.3,350.));
#6438=CARTESIAN_POINT('',(-198.,-111.3,350.));
#6439=CARTESIAN_POINT('',(-198.,0.,350.));
#6440=CARTESIAN_POINT('',(-4.28626379701574E-14,-111.3,350.));
#6441=CARTESIAN_POINT('Origin',(-4.24952439304132E-14,-111.3,347.));
#6442=CARTESIAN_POINT('',(-198.,-114.3,347.));
#6443=CARTESIAN_POINT('Origin',(-198.,-111.3,347.));
#6444=CARTESIAN_POINT('',(-4.24952439304132E-14,-114.3,347.));
#6445=CARTESIAN_POINT('Origin',(-3.95560916124595E-14,-114.3,323.));
#6446=CARTESIAN_POINT('',(-198.,-114.3,323.));
#6447=CARTESIAN_POINT('',(-198.,-114.3,347.));
#6448=CARTESIAN_POINT('',(-3.95560916124595E-14,-114.3,323.));
#6449=CARTESIAN_POINT('Origin',(-3.95560916124595E-14,-111.3,323.));
#6450=CARTESIAN_POINT('',(-198.,-111.3,320.));
#6451=CARTESIAN_POINT('Origin',(-198.,-111.3,323.));
#6452=CARTESIAN_POINT('',(-3.91886975727153E-14,-111.3,320.));
#6453=CARTESIAN_POINT('Origin',(-3.91886975727153E-14,-99.3,320.));
#6454=CARTESIAN_POINT('',(-198.,-111.3,320.));
#6455=CARTESIAN_POINT('Origin',(-198.,-57.15,335.));
#74508=UNCERTAINTY_MEASURE_WITH_UNIT(LENGTH_MEASURE(0.01),#74524,
'DISTANCE_ACCURACY_VALUE',
'Maximum model space distance between geometric entities at asserted c
onnectivities');
#74512=UNCERTAINTY_MEASURE_WITH_UNIT(LENGTH_MEASURE(0.01),#74524,
'DISTANCE_ACCURACY_VALUE',
'Maximum model space distance between geometric entities at asserted c
onnectivities');
#74519=(
GEOMETRIC_REPRESENTATION_CONTEXT(3)
GLOBAL_UNCERTAINTY_ASSIGNED_CONTEXT((#74508))
GLOBAL_UNIT_ASSIGNED_CONTEXT((#74524,#74526,#74527))
REPRESENTATION_CONTEXT('','3D')
);
#74523=(
GEOMETRIC_REPRESENTATION_CONTEXT(3)
GLOBAL_UNCERTAINTY_ASSIGNED_CONTEXT((#74512))
GLOBAL_UNIT_ASSIGNED_CONTEXT((#74524,#74526,#74527))
REPRESENTATION_CONTEXT('','3D')
);
#74524=(
LENGTH_UNIT()
NAMED_UNIT(*)
SI_UNIT(.MILLI.,.METRE.)
);
#74526=(
NAMED_UNIT(*)
PLANE_ANGLE_UNIT()
SI_UNIT($,.RADIAN.)
);
#74527=(
NAMED_UNIT(*)
SI_UNIT($,.STERADIAN.)
SOLID_ANGLE_UNIT()
);
#74534=SHAPE_DEFINITION_REPRESENTATION(#74544,#74563);
#74544=PRODUCT_DEFINITION_SHAPE('',$,#74574);
#74563=SHAPE_REPRESENTATION('',(#4986),#74519);
#74567=PRODUCT_DEFINITION_CONTEXT('part definition',#74599,'design');
#74574=PRODUCT_DEFINITION('Top_Base','Top_Base',#74584,#74567);
#74584=PRODUCT_DEFINITION_FORMATION('',$,#74607);
#74599=APPLICATION_CONTEXT(
'Core Data for Automotive Mechanical Design Process');
#74600=PRODUCT_CONTEXT('part definition',#74599,'mechanical');
#74607=PRODUCT('Top_Base','Top_Base',$,(#74600));
#74612=PRESENTATION_STYLE_ASSIGNMENT((#74615));
#74615=SURFACE_STYLE_USAGE(.BOTH.,#74618);
#74618=SURFACE_SIDE_STYLE('',(#74621));
#74621=SURFACE_STYLE_FILL_AREA(#74624);
#74624=FILL_AREA_STYLE('Opaque(215,0,0)',(#74627));
#74627=FILL_AREA_STYLE_COLOUR('Opaque(215,0,0)',#74630);
#74630=COLOUR_RGB('Opaque(215,0,0)', 0.09019608, 0.27058824, 0.51372549);
ENDSEC;
END-ISO-10303-21;
